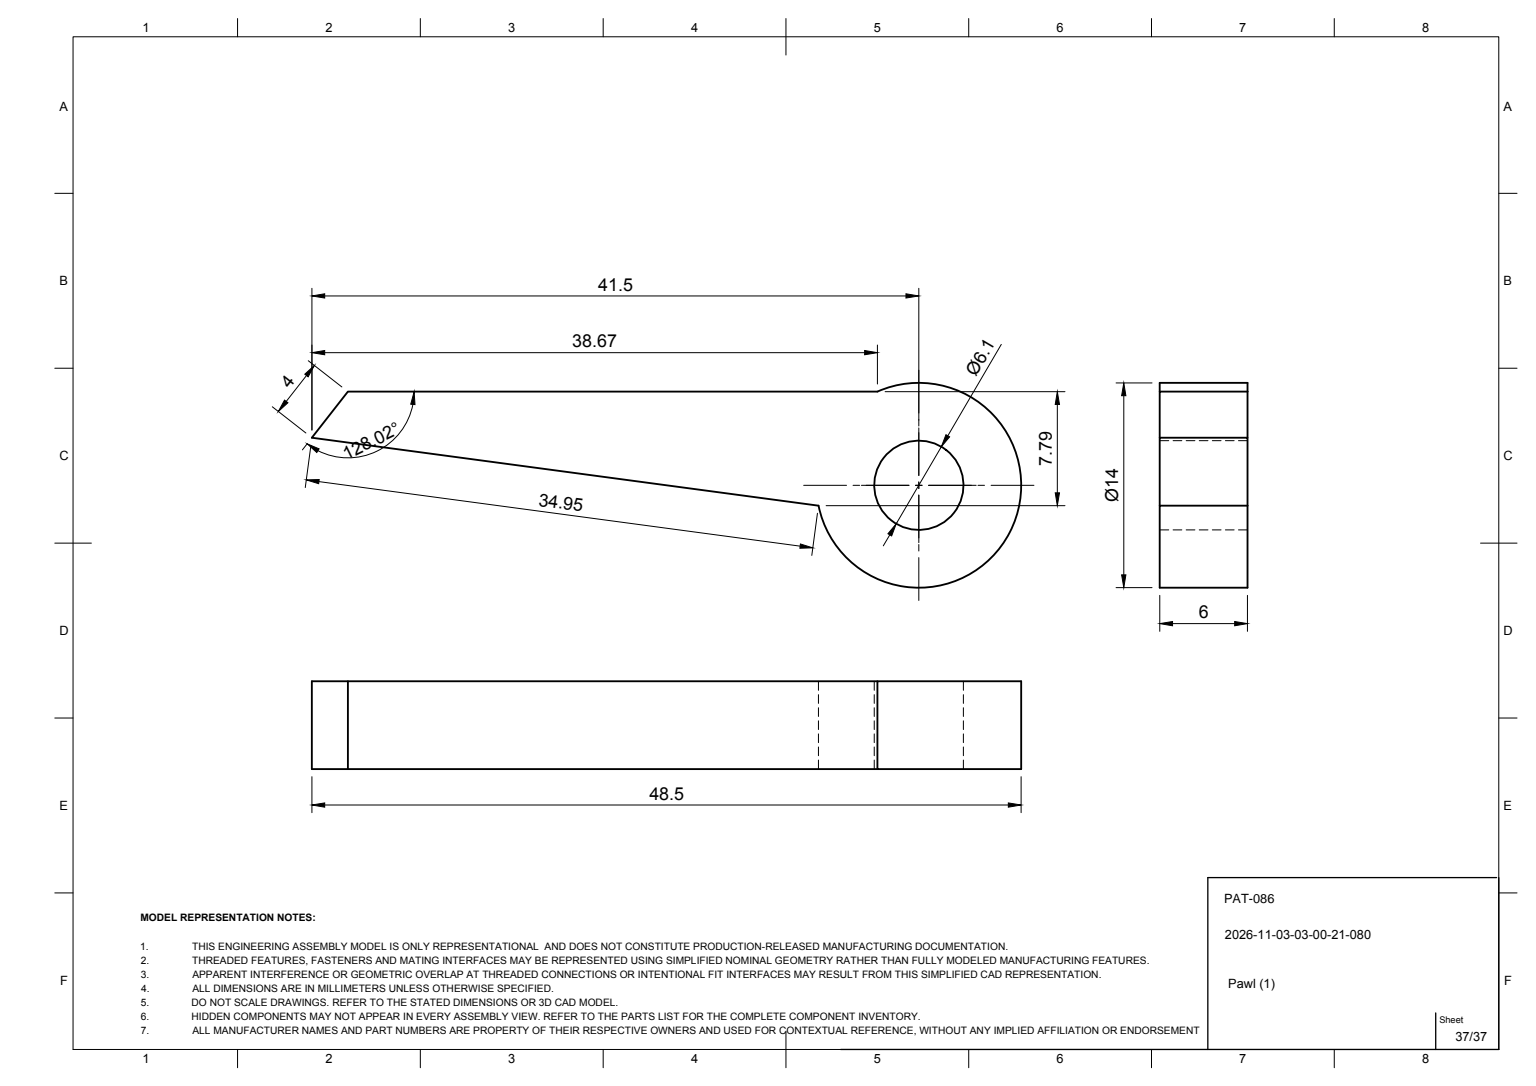
ISO-10303-21;
HEADER;
/* Generated by software containing ST-Developer
 * from STEP Tools, Inc. (www.steptools.com) 
 */

FILE_DESCRIPTION(
/* description */ ('Ratchet and pawl hand winch drum'),
/* implementation_level */ '2;1');

FILE_NAME(
/* name */ 'Pawl (1).step',
/* time_stamp */ '2026-10-27T12:42:58-07:00',
/* author */ (''),
/* organization */ (''),
/* preprocessor_version */ 'ST-DEVELOPER v20.2',
/* originating_system */ 'Autodesk Translation Framework v15.17.0.0',
/* authorisation */ '');

FILE_SCHEMA (('AUTOMOTIVE_DESIGN { 1 0 10303 214 3 1 1 }'));
ENDSEC;

DATA;
#10=MECHANICAL_DESIGN_GEOMETRIC_PRESENTATION_REPRESENTATION('',(#423),#11801);
#354=SHAPE_REPRESENTATION_RELATIONSHIP('SRR','None',#11983,#388);
#388=ADVANCED_BREP_SHAPE_REPRESENTATION('',(#455),#11800);
#423=STYLED_ITEM('',(#12199),#455);
#455=MANIFOLD_SOLID_BREP('Body1',#6303);
#599=FACE_BOUND('',#1692,.T.);
#600=FACE_BOUND('',#1696,.T.);
#835=PLANE('',#7349);
#836=PLANE('',#7350);
#837=PLANE('',#7351);
#838=PLANE('',#7352);
#839=PLANE('',#7353);
#1189=FACE_OUTER_BOUND('',#1688,.T.);
#1190=FACE_OUTER_BOUND('',#1689,.T.);
#1191=FACE_OUTER_BOUND('',#1690,.T.);
#1192=FACE_OUTER_BOUND('',#1691,.T.);
#1193=FACE_OUTER_BOUND('',#1693,.T.);
#1194=FACE_OUTER_BOUND('',#1694,.T.);
#1195=FACE_OUTER_BOUND('',#1695,.T.);
#1688=EDGE_LOOP('',(#5777,#5778,#5779,#5780));
#1689=EDGE_LOOP('',(#5781,#5782,#5783,#5784));
#1690=EDGE_LOOP('',(#5785,#5786,#5787,#5788));
#1691=EDGE_LOOP('',(#5789,#5790,#5791,#5792));
#1692=EDGE_LOOP('',(#5793));
#1693=EDGE_LOOP('',(#5794,#5795,#5796,#5797));
#1694=EDGE_LOOP('',(#5798,#5799,#5800,#5801));
#1695=EDGE_LOOP('',(#5802,#5803,#5804,#5805));
#1696=EDGE_LOOP('',(#5806));
#2197=LINE('',#11690,#2708);
#2198=LINE('',#11695,#2709);
#2199=LINE('',#11699,#2710);
#2200=LINE('',#11703,#2711);
#2201=LINE('',#11705,#2712);
#2202=LINE('',#11706,#2713);
#2203=LINE('',#11709,#2714);
#2204=LINE('',#11710,#2715);
#2205=LINE('',#11713,#2716);
#2206=LINE('',#11714,#2717);
#2207=LINE('',#11716,#2718);
#2708=VECTOR('',#9190,0.305);
#2709=VECTOR('',#9195,1.);
#2710=VECTOR('',#9198,1.);
#2711=VECTOR('',#9203,1.);
#2712=VECTOR('',#9204,1.);
#2713=VECTOR('',#9205,1.);
#2714=VECTOR('',#9208,1.);
#2715=VECTOR('',#9209,1.);
#2716=VECTOR('',#9212,1.);
#2717=VECTOR('',#9213,1.);
#2718=VECTOR('',#9216,1.);
#2938=CIRCLE('',#7344,0.305);
#2939=CIRCLE('',#7345,0.305);
#2940=CIRCLE('',#7347,0.7);
#2941=CIRCLE('',#7348,0.7);
#3457=VERTEX_POINT('',#11687);
#3458=VERTEX_POINT('',#11689);
#3459=VERTEX_POINT('',#11693);
#3460=VERTEX_POINT('',#11694);
#3461=VERTEX_POINT('',#11696);
#3462=VERTEX_POINT('',#11698);
#3463=VERTEX_POINT('',#11702);
#3464=VERTEX_POINT('',#11704);
#3465=VERTEX_POINT('',#11708);
#3466=VERTEX_POINT('',#11712);
#4232=EDGE_CURVE('',#3457,#3457,#2938,.T.);
#4233=EDGE_CURVE('',#3457,#3458,#2197,.T.);
#4234=EDGE_CURVE('',#3458,#3458,#2939,.T.);
#4235=EDGE_CURVE('',#3459,#3460,#2198,.T.);
#4236=EDGE_CURVE('',#3459,#3461,#2940,.T.);
#4237=EDGE_CURVE('',#3462,#3461,#2199,.T.);
#4238=EDGE_CURVE('',#3460,#3462,#2941,.T.);
#4239=EDGE_CURVE('',#3463,#3460,#2200,.T.);
#4240=EDGE_CURVE('',#3464,#3463,#2201,.T.);
#4241=EDGE_CURVE('',#3459,#3464,#2202,.T.);
#4242=EDGE_CURVE('',#3462,#3465,#2203,.T.);
#4243=EDGE_CURVE('',#3465,#3463,#2204,.T.);
#4244=EDGE_CURVE('',#3464,#3466,#2205,.T.);
#4245=EDGE_CURVE('',#3466,#3465,#2206,.T.);
#4246=EDGE_CURVE('',#3466,#3461,#2207,.T.);
#5777=ORIENTED_EDGE('',*,*,#4232,.F.);
#5778=ORIENTED_EDGE('',*,*,#4233,.T.);
#5779=ORIENTED_EDGE('',*,*,#4234,.F.);
#5780=ORIENTED_EDGE('',*,*,#4233,.F.);
#5781=ORIENTED_EDGE('',*,*,#4235,.F.);
#5782=ORIENTED_EDGE('',*,*,#4236,.T.);
#5783=ORIENTED_EDGE('',*,*,#4237,.F.);
#5784=ORIENTED_EDGE('',*,*,#4238,.F.);
#5785=ORIENTED_EDGE('',*,*,#4235,.T.);
#5786=ORIENTED_EDGE('',*,*,#4239,.F.);
#5787=ORIENTED_EDGE('',*,*,#4240,.F.);
#5788=ORIENTED_EDGE('',*,*,#4241,.F.);
#5789=ORIENTED_EDGE('',*,*,#4238,.T.);
#5790=ORIENTED_EDGE('',*,*,#4242,.T.);
#5791=ORIENTED_EDGE('',*,*,#4243,.T.);
#5792=ORIENTED_EDGE('',*,*,#4239,.T.);
#5793=ORIENTED_EDGE('',*,*,#4234,.T.);
#5794=ORIENTED_EDGE('',*,*,#4244,.F.);
#5795=ORIENTED_EDGE('',*,*,#4240,.T.);
#5796=ORIENTED_EDGE('',*,*,#4243,.F.);
#5797=ORIENTED_EDGE('',*,*,#4245,.F.);
#5798=ORIENTED_EDGE('',*,*,#4237,.T.);
#5799=ORIENTED_EDGE('',*,*,#4246,.F.);
#5800=ORIENTED_EDGE('',*,*,#4245,.T.);
#5801=ORIENTED_EDGE('',*,*,#4242,.F.);
#5802=ORIENTED_EDGE('',*,*,#4241,.T.);
#5803=ORIENTED_EDGE('',*,*,#4244,.T.);
#5804=ORIENTED_EDGE('',*,*,#4246,.T.);
#5805=ORIENTED_EDGE('',*,*,#4236,.F.);
#5806=ORIENTED_EDGE('',*,*,#4232,.T.);
#5908=CYLINDRICAL_SURFACE('',#7343,0.305);
#5909=CYLINDRICAL_SURFACE('',#7346,0.7);
#6259=ADVANCED_FACE('',(#1189),#5908,.F.);
#6260=ADVANCED_FACE('',(#1190),#5909,.T.);
#6261=ADVANCED_FACE('',(#1191),#835,.T.);
#6262=ADVANCED_FACE('',(#1192,#599),#836,.T.);
#6263=ADVANCED_FACE('',(#1193),#837,.T.);
#6264=ADVANCED_FACE('',(#1194),#838,.T.);
#6265=ADVANCED_FACE('',(#1195,#600),#839,.F.);
#6303=CLOSED_SHELL('',(#6259,#6260,#6261,#6262,#6263,#6264,#6265));
#7342=AXIS2_PLACEMENT_3D('',#11685,#9184,#9185);
#7343=AXIS2_PLACEMENT_3D('',#11686,#9186,#9187);
#7344=AXIS2_PLACEMENT_3D('',#11688,#9188,#9189);
#7345=AXIS2_PLACEMENT_3D('',#11691,#9191,#9192);
#7346=AXIS2_PLACEMENT_3D('',#11692,#9193,#9194);
#7347=AXIS2_PLACEMENT_3D('',#11697,#9196,#9197);
#7348=AXIS2_PLACEMENT_3D('',#11700,#9199,#9200);
#7349=AXIS2_PLACEMENT_3D('',#11701,#9201,#9202);
#7350=AXIS2_PLACEMENT_3D('',#11707,#9206,#9207);
#7351=AXIS2_PLACEMENT_3D('',#11711,#9210,#9211);
#7352=AXIS2_PLACEMENT_3D('',#11715,#9214,#9215);
#7353=AXIS2_PLACEMENT_3D('',#11717,#9217,#9218);
#9184=DIRECTION('axis',(0.,0.,1.));
#9185=DIRECTION('refdir',(1.,0.,0.));
#9186=DIRECTION('center_axis',(0.,1.,0.));
#9187=DIRECTION('ref_axis',(1.,0.,0.));
#9188=DIRECTION('center_axis',(0.,1.,0.));
#9189=DIRECTION('ref_axis',(1.,0.,0.));
#9190=DIRECTION('',(0.,1.,0.));
#9191=DIRECTION('center_axis',(0.,-1.,0.));
#9192=DIRECTION('ref_axis',(1.,0.,0.));
#9193=DIRECTION('center_axis',(0.,1.,0.));
#9194=DIRECTION('ref_axis',(0.185131832090925,0.,0.982713694189034));
#9195=DIRECTION('',(0.,1.,0.));
#9196=DIRECTION('center_axis',(0.,1.,0.));
#9197=DIRECTION('ref_axis',(1.,0.,0.));
#9198=DIRECTION('',(0.,-1.,0.));
#9199=DIRECTION('center_axis',(0.,1.,0.));
#9200=DIRECTION('ref_axis',(1.,0.,0.));
#9201=DIRECTION('center_axis',(-0.862655693448417,0.,0.50579161179386));
#9202=DIRECTION('ref_axis',(0.50579161179386,0.,0.862655693448417));
#9203=DIRECTION('',(0.50579161179386,0.,0.862655693448417));
#9204=DIRECTION('',(0.,1.,0.));
#9205=DIRECTION('',(-0.50579161179386,0.,-0.862655693448417));
#9206=DIRECTION('center_axis',(0.,1.,0.));
#9207=DIRECTION('ref_axis',(0.,0.,1.));
#9208=DIRECTION('',(-0.615893007805892,0.,-0.78782980581837));
#9209=DIRECTION('',(-1.,0.,0.));
#9210=DIRECTION('center_axis',(0.,0.,-1.));
#9211=DIRECTION('ref_axis',(-1.,0.,0.));
#9212=DIRECTION('',(1.,0.,0.));
#9213=DIRECTION('',(0.,1.,0.));
#9214=DIRECTION('center_axis',(0.78782980581837,0.,-0.615893007805892));
#9215=DIRECTION('ref_axis',(-0.615893007805892,0.,-0.78782980581837));
#9216=DIRECTION('',(0.615893007805892,0.,0.78782980581837));
#9217=DIRECTION('center_axis',(0.,1.,0.));
#9218=DIRECTION('ref_axis',(1.,0.,0.));
#11685=CARTESIAN_POINT('',(0.,0.,0.));
#11686=CARTESIAN_POINT('Origin',(6.5,-3.6,10.));
#11687=CARTESIAN_POINT('',(6.195,-3.5,10.));
#11688=CARTESIAN_POINT('Origin',(6.5,-3.5,10.));
#11689=CARTESIAN_POINT('',(6.195,-2.9,10.));
#11690=CARTESIAN_POINT('',(6.195,-3.6,10.));
#11691=CARTESIAN_POINT('Origin',(6.5,-2.9,10.));
#11692=CARTESIAN_POINT('Origin',(6.5,-3.5,10.));
#11693=CARTESIAN_POINT('',(5.96787188180707,-3.5,9.54520370952651));
#11694=CARTESIAN_POINT('',(5.96787188180707,-2.9,9.54520370952651));
#11695=CARTESIAN_POINT('',(5.96787188180707,-3.5,9.54520370952651));
#11696=CARTESIAN_POINT('',(6.83016839641497,-3.5,9.38275707374749));
#11697=CARTESIAN_POINT('Origin',(6.5,-3.5,10.));
#11698=CARTESIAN_POINT('',(6.83016839641497,-2.9,9.38275707374749));
#11699=CARTESIAN_POINT('',(6.83016839641497,-3.5,9.38275707374749));
#11700=CARTESIAN_POINT('Origin',(6.5,-2.9,10.));
#11701=CARTESIAN_POINT('Origin',(4.2,-3.5,6.53));
#11702=CARTESIAN_POINT('',(4.2,-2.9,6.53));
#11703=CARTESIAN_POINT('',(6.,-2.9,9.6));
#11704=CARTESIAN_POINT('',(4.2,-3.5,6.53));
#11705=CARTESIAN_POINT('',(4.2,-3.5,6.53));
#11706=CARTESIAN_POINT('',(6.,-3.5,9.6));
#11707=CARTESIAN_POINT('Origin',(5.6,-2.9,8.465));
#11708=CARTESIAN_POINT('',(4.6,-2.9,6.53));
#11709=CARTESIAN_POINT('',(4.6,-2.9,6.53));
#11710=CARTESIAN_POINT('',(4.2,-2.9,6.53));
#11711=CARTESIAN_POINT('Origin',(4.6,-3.5,6.53));
#11712=CARTESIAN_POINT('',(4.6,-3.5,6.53));
#11713=CARTESIAN_POINT('',(4.2,-3.5,6.53));
#11714=CARTESIAN_POINT('',(4.6,-3.5,6.53));
#11715=CARTESIAN_POINT('Origin',(7.,-3.5,9.6));
#11716=CARTESIAN_POINT('',(4.6,-3.5,6.53));
#11717=CARTESIAN_POINT('Origin',(5.6,-3.5,8.465));
#11760=UNCERTAINTY_MEASURE_WITH_UNIT(LENGTH_MEASURE(0.001),#11802,
'DISTANCE_ACCURACY_VALUE',
'Maximum model space distance between geometric entities at asserted c
onnectivities');
#11761=UNCERTAINTY_MEASURE_WITH_UNIT(LENGTH_MEASURE(0.001),#11802,
'DISTANCE_ACCURACY_VALUE',
'Maximum model space distance between geometric entities at asserted c
onnectivities');
#11800=(
GEOMETRIC_REPRESENTATION_CONTEXT(3)
GLOBAL_UNCERTAINTY_ASSIGNED_CONTEXT((#11760))
GLOBAL_UNIT_ASSIGNED_CONTEXT((#11802,#11804,#11805))
REPRESENTATION_CONTEXT('','3D')
);
#11801=(
GEOMETRIC_REPRESENTATION_CONTEXT(3)
GLOBAL_UNCERTAINTY_ASSIGNED_CONTEXT((#11761))
GLOBAL_UNIT_ASSIGNED_CONTEXT((#11802,#11804,#11805))
REPRESENTATION_CONTEXT('','3D')
);
#11802=(
LENGTH_UNIT()
NAMED_UNIT(*)
SI_UNIT(.CENTI.,.METRE.)
);
#11804=(
NAMED_UNIT(*)
PLANE_ANGLE_UNIT()
SI_UNIT($,.RADIAN.)
);
#11805=(
NAMED_UNIT(*)
SI_UNIT($,.STERADIAN.)
SOLID_ANGLE_UNIT()
);
#11844=SHAPE_DEFINITION_REPRESENTATION(#11940,#11983);
#11940=PRODUCT_DEFINITION_SHAPE('',$,#12023);
#11983=SHAPE_REPRESENTATION('',(#7342),#11800);
#11984=PRODUCT_DEFINITION_CONTEXT('part definition',#12103,'design');
#12023=PRODUCT_DEFINITION('Pawl (1)','Pawl (1)',#12062,#11984);
#12062=PRODUCT_DEFINITION_FORMATION('',$,#12143);
#12103=APPLICATION_CONTEXT(
'Core Data for Automotive Mechanical Design Process');
#12104=PRODUCT_CONTEXT('part definition',#12103,'mechanical');
#12143=PRODUCT('Pawl (1)','Pawl (1)','Pawl (1)',(#12104));
#12193=COLOUR_RGB('Light Blue',0.38,0.62,0.78);
#12194=FILL_AREA_STYLE_COLOUR('',#12193);
#12195=FILL_AREA_STYLE('',(#12194));
#12196=SURFACE_STYLE_FILL_AREA(#12195);
#12197=SURFACE_SIDE_STYLE('',(#12196));
#12198=SURFACE_STYLE_USAGE(.BOTH.,#12197);
#12199=PRESENTATION_STYLE_ASSIGNMENT((#12198));
ENDSEC;
END-ISO-10303-21;
